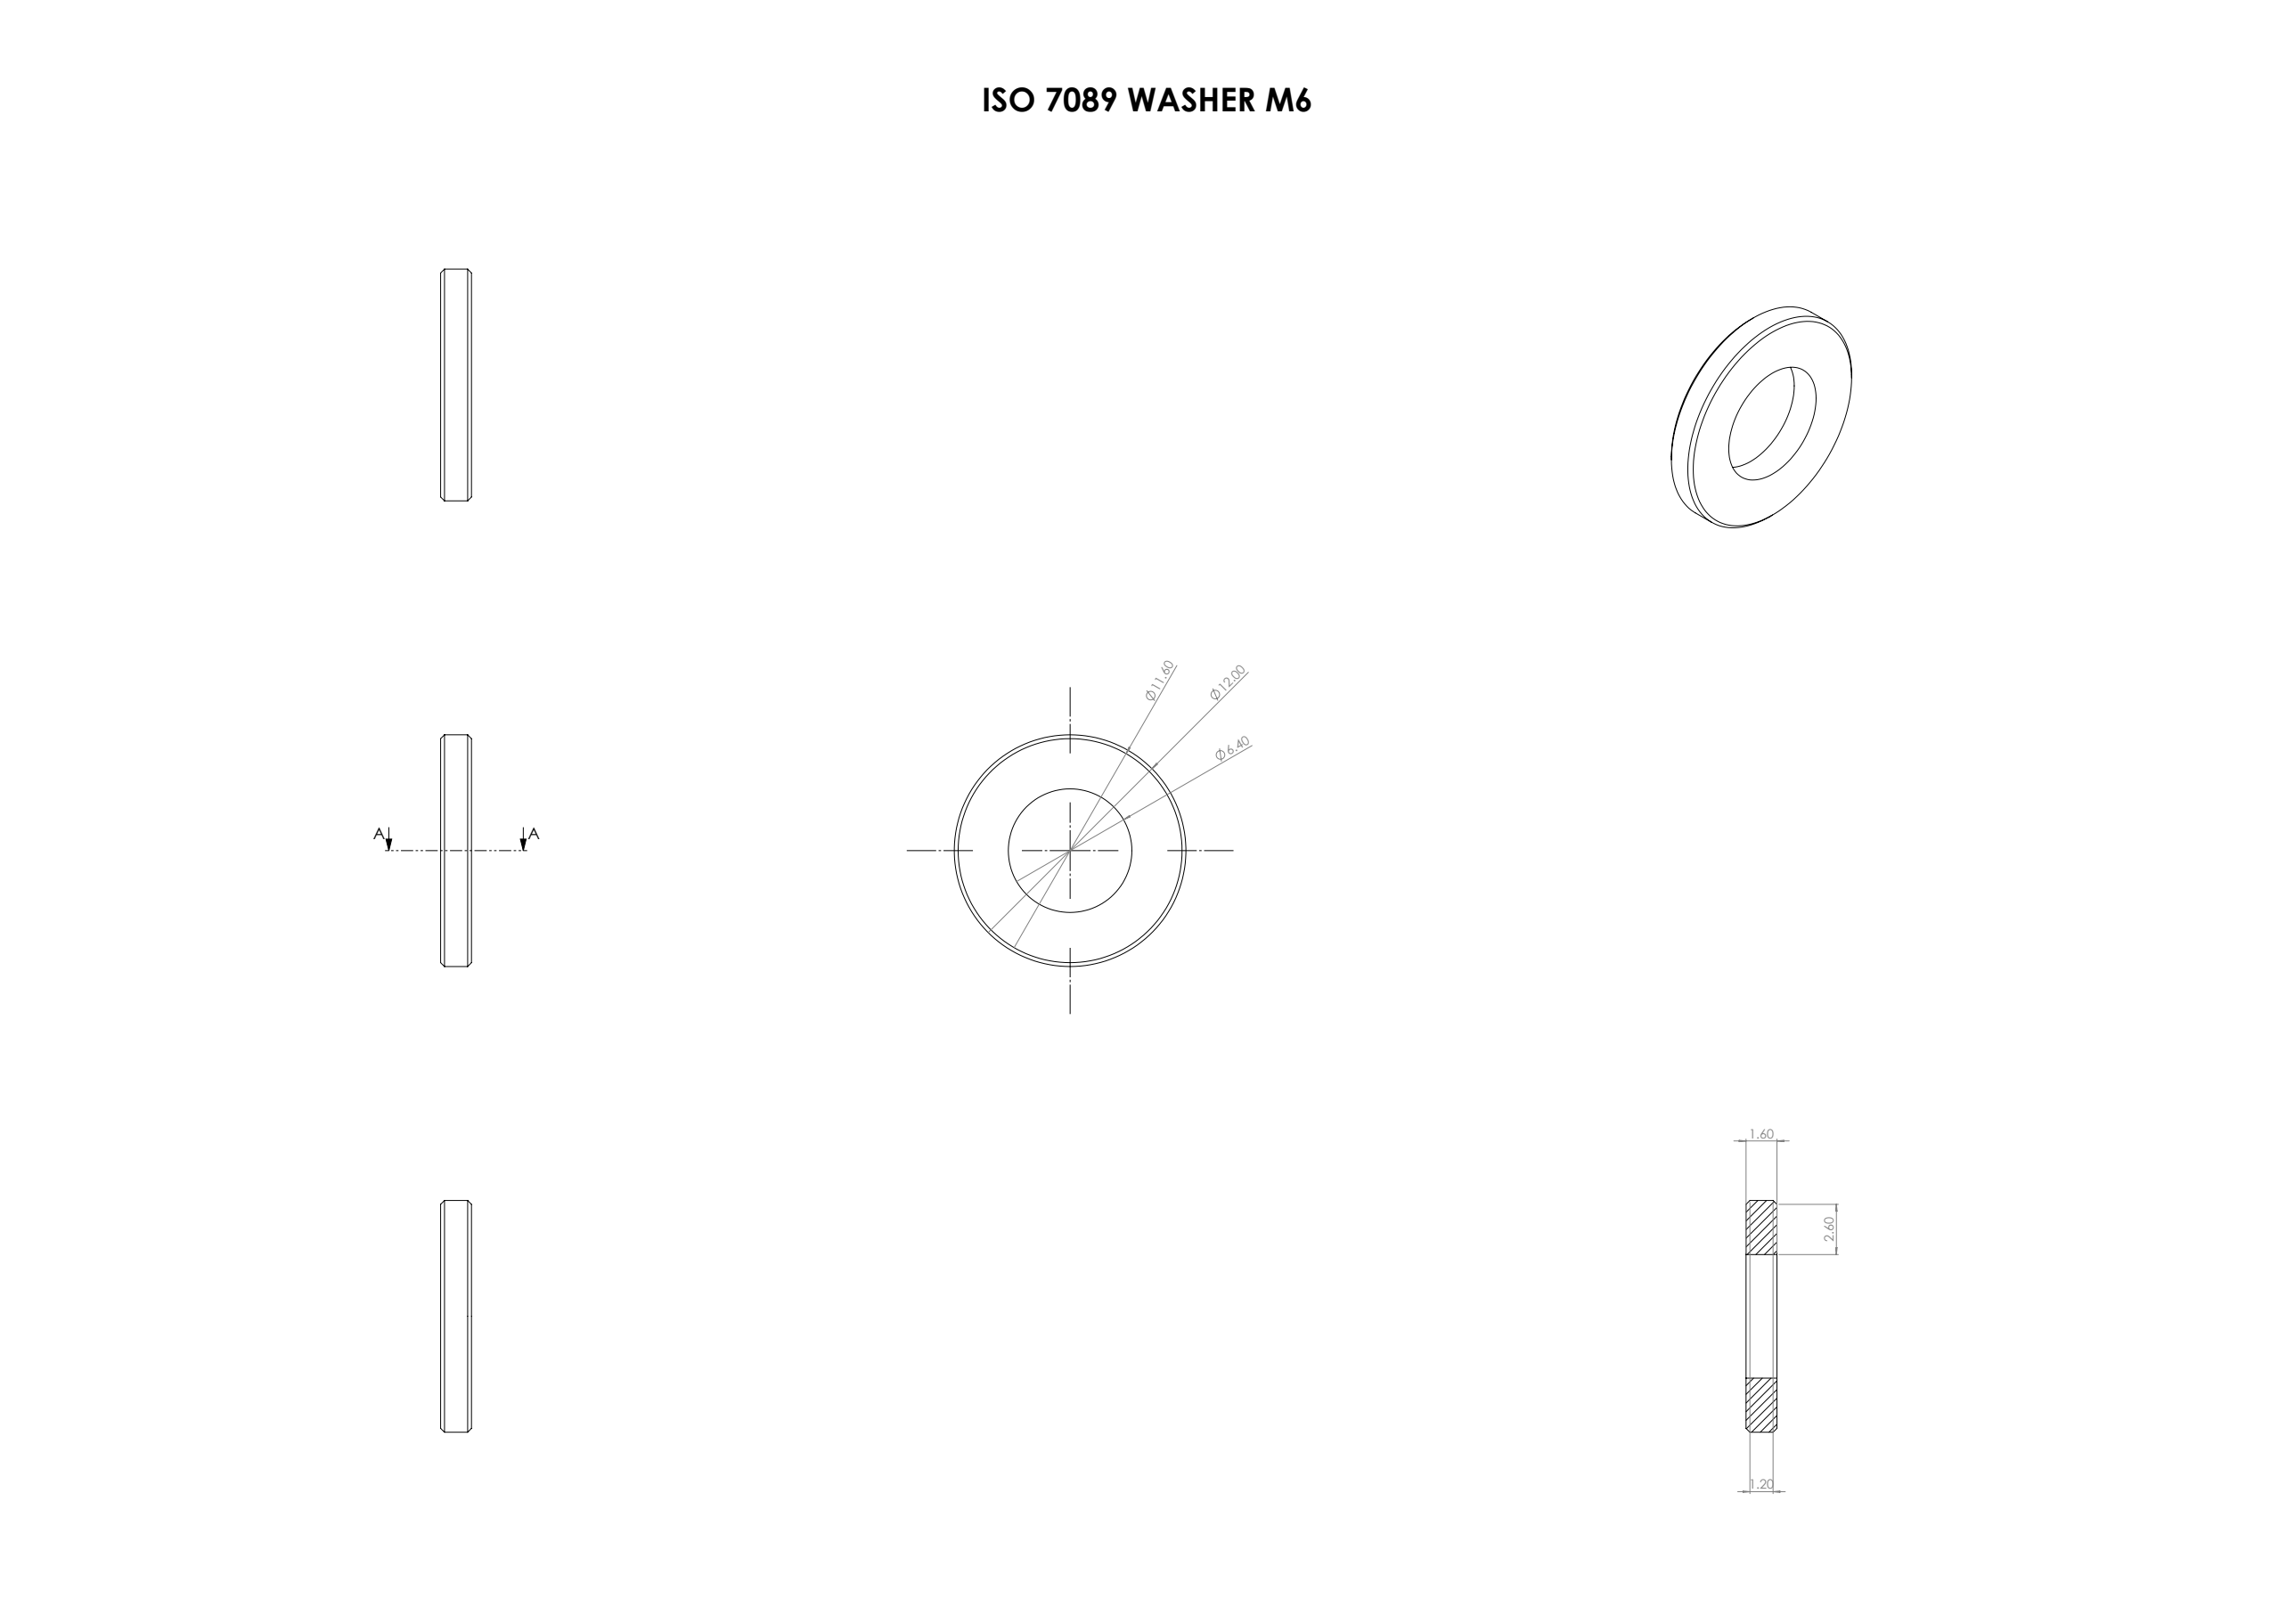
ISO-10303-21;
HEADER;
/* Generated by software containing ST-Developer
 * from STEP Tools, Inc. (www.steptools.com) 
 */

FILE_DESCRIPTION(
/* description */ (''),
/* implementation_level */ '2;1');

FILE_NAME(
/* name */ '07_ISO_7089_Washer_M6.step',
/* time_stamp */ '2026-10-21T02:03:06-07:00',
/* author */ (''),
/* organization */ (''),
/* preprocessor_version */ 'ST-DEVELOPER v20.2',
/* originating_system */ 'Autodesk Translation Framework v15.15.0.0',
/* authorisation */ '');

FILE_SCHEMA (('AUTOMOTIVE_DESIGN { 1 0 10303 214 3 1 1 }'));
ENDSEC;

DATA;
#10=MECHANICAL_DESIGN_GEOMETRIC_PRESENTATION_REPRESENTATION('',(#121),#38528);
#97=SHAPE_REPRESENTATION_RELATIONSHIP('SRR','None',#38582,#109);
#109=ADVANCED_BREP_SHAPE_REPRESENTATION('',(#133),#38522);
#121=STYLED_ITEM('',(#38713),#133);
#133=MANIFOLD_SOLID_BREP('Body1',#17078);
#383=CYLINDRICAL_SURFACE('',#18713,6.);
#384=CYLINDRICAL_SURFACE('',#18717,3.2);
#1034=CONICAL_SURFACE('',#18709,5.9,0.785398163397449);
#1035=CONICAL_SURFACE('',#18721,5.9,0.785398163397449);
#1471=FACE_BOUND('',#4085,.T.);
#1472=FACE_BOUND('',#4088,.T.);
#2177=CIRCLE('',#18710,5.8);
#2178=CIRCLE('',#18711,6.);
#2179=CIRCLE('',#18712,6.);
#2180=CIRCLE('',#18714,6.);
#2181=CIRCLE('',#18716,3.2);
#2182=CIRCLE('',#18718,3.2);
#2183=CIRCLE('',#18720,5.8);
#3060=FACE_OUTER_BOUND('',#4082,.T.);
#3061=FACE_OUTER_BOUND('',#4083,.T.);
#3062=FACE_OUTER_BOUND('',#4084,.T.);
#3063=FACE_OUTER_BOUND('',#4086,.T.);
#3064=FACE_OUTER_BOUND('',#4087,.T.);
#3065=FACE_OUTER_BOUND('',#4089,.T.);
#4082=EDGE_LOOP('',(#14531,#14532,#14533,#14534,#14535));
#4083=EDGE_LOOP('',(#14536,#14537,#14538,#14539,#14540));
#4084=EDGE_LOOP('',(#14541));
#4085=EDGE_LOOP('',(#14542));
#4086=EDGE_LOOP('',(#14543,#14544,#14545,#14546));
#4087=EDGE_LOOP('',(#14547));
#4088=EDGE_LOOP('',(#14548));
#4089=EDGE_LOOP('',(#14549,#14550,#14551,#14552));
#5028=LINE('',#33185,#6003);
#5029=LINE('',#33191,#6004);
#5030=LINE('',#33198,#6005);
#5031=LINE('',#33204,#6006);
#6003=VECTOR('',#22750,5.9);
#6004=VECTOR('',#22757,6.);
#6005=VECTOR('',#22766,3.2);
#6006=VECTOR('',#22775,5.9);
#7528=VERTEX_POINT('',#33182);
#7529=VERTEX_POINT('',#33184);
#7530=VERTEX_POINT('',#33186);
#7531=VERTEX_POINT('',#33190);
#7532=VERTEX_POINT('',#33194);
#7533=VERTEX_POINT('',#33197);
#7534=VERTEX_POINT('',#33201);
#9917=EDGE_CURVE('',#7528,#7528,#2177,.T.);
#9918=EDGE_CURVE('',#7528,#7529,#5028,.T.);
#9919=EDGE_CURVE('',#7529,#7530,#2178,.T.);
#9920=EDGE_CURVE('',#7530,#7529,#2179,.T.);
#9921=EDGE_CURVE('',#7530,#7531,#5029,.T.);
#9922=EDGE_CURVE('',#7531,#7531,#2180,.T.);
#9923=EDGE_CURVE('',#7532,#7532,#2181,.T.);
#9924=EDGE_CURVE('',#7532,#7533,#5030,.T.);
#9925=EDGE_CURVE('',#7533,#7533,#2182,.T.);
#9926=EDGE_CURVE('',#7534,#7534,#2183,.T.);
#9927=EDGE_CURVE('',#7531,#7534,#5031,.T.);
#14531=ORIENTED_EDGE('',*,*,#9917,.T.);
#14532=ORIENTED_EDGE('',*,*,#9918,.T.);
#14533=ORIENTED_EDGE('',*,*,#9919,.T.);
#14534=ORIENTED_EDGE('',*,*,#9920,.T.);
#14535=ORIENTED_EDGE('',*,*,#9918,.F.);
#14536=ORIENTED_EDGE('',*,*,#9919,.F.);
#14537=ORIENTED_EDGE('',*,*,#9920,.F.);
#14538=ORIENTED_EDGE('',*,*,#9921,.T.);
#14539=ORIENTED_EDGE('',*,*,#9922,.T.);
#14540=ORIENTED_EDGE('',*,*,#9921,.F.);
#14541=ORIENTED_EDGE('',*,*,#9917,.F.);
#14542=ORIENTED_EDGE('',*,*,#9923,.F.);
#14543=ORIENTED_EDGE('',*,*,#9923,.T.);
#14544=ORIENTED_EDGE('',*,*,#9924,.T.);
#14545=ORIENTED_EDGE('',*,*,#9925,.F.);
#14546=ORIENTED_EDGE('',*,*,#9924,.F.);
#14547=ORIENTED_EDGE('',*,*,#9926,.F.);
#14548=ORIENTED_EDGE('',*,*,#9925,.T.);
#14549=ORIENTED_EDGE('',*,*,#9922,.F.);
#14550=ORIENTED_EDGE('',*,*,#9927,.T.);
#14551=ORIENTED_EDGE('',*,*,#9926,.T.);
#14552=ORIENTED_EDGE('',*,*,#9927,.F.);
#15960=PLANE('',#18715);
#15961=PLANE('',#18719);
#16869=ADVANCED_FACE('',(#3060),#1034,.T.);
#16870=ADVANCED_FACE('',(#3061),#383,.T.);
#16871=ADVANCED_FACE('',(#3062,#1471),#15960,.T.);
#16872=ADVANCED_FACE('',(#3063),#384,.F.);
#16873=ADVANCED_FACE('',(#3064,#1472),#15961,.T.);
#16874=ADVANCED_FACE('',(#3065),#1035,.T.);
#17078=CLOSED_SHELL('',(#16869,#16870,#16871,#16872,#16873,#16874));
#18708=AXIS2_PLACEMENT_3D('',#33180,#22744,#22745);
#18709=AXIS2_PLACEMENT_3D('',#33181,#22746,#22747);
#18710=AXIS2_PLACEMENT_3D('',#33183,#22748,#22749);
#18711=AXIS2_PLACEMENT_3D('',#33187,#22751,#22752);
#18712=AXIS2_PLACEMENT_3D('',#33188,#22753,#22754);
#18713=AXIS2_PLACEMENT_3D('',#33189,#22755,#22756);
#18714=AXIS2_PLACEMENT_3D('',#33192,#22758,#22759);
#18715=AXIS2_PLACEMENT_3D('',#33193,#22760,#22761);
#18716=AXIS2_PLACEMENT_3D('',#33195,#22762,#22763);
#18717=AXIS2_PLACEMENT_3D('',#33196,#22764,#22765);
#18718=AXIS2_PLACEMENT_3D('',#33199,#22767,#22768);
#18719=AXIS2_PLACEMENT_3D('',#33200,#22769,#22770);
#18720=AXIS2_PLACEMENT_3D('',#33202,#22771,#22772);
#18721=AXIS2_PLACEMENT_3D('',#33203,#22773,#22774);
#22744=DIRECTION('axis',(0.,0.,1.));
#22745=DIRECTION('refdir',(1.,0.,0.));
#22746=DIRECTION('center_axis',(-1.,0.,0.));
#22747=DIRECTION('ref_axis',(0.,-1.,0.));
#22748=DIRECTION('center_axis',(-1.,0.,0.));
#22749=DIRECTION('ref_axis',(0.,-1.,0.));
#22750=DIRECTION('',(-0.707106781186547,0.707106781186548,8.65956056235494E-17));
#22751=DIRECTION('center_axis',(1.,0.,0.));
#22752=DIRECTION('ref_axis',(0.,-1.,0.));
#22753=DIRECTION('center_axis',(1.,0.,0.));
#22754=DIRECTION('ref_axis',(0.,-1.,0.));
#22755=DIRECTION('center_axis',(1.,0.,0.));
#22756=DIRECTION('ref_axis',(0.,1.,0.));
#22757=DIRECTION('',(-1.,0.,0.));
#22758=DIRECTION('center_axis',(1.,0.,0.));
#22759=DIRECTION('ref_axis',(0.,0.,-1.));
#22760=DIRECTION('center_axis',(1.,0.,0.));
#22761=DIRECTION('ref_axis',(0.,0.,-1.));
#22762=DIRECTION('center_axis',(1.,0.,0.));
#22763=DIRECTION('ref_axis',(0.,0.,-1.));
#22764=DIRECTION('center_axis',(1.,0.,0.));
#22765=DIRECTION('ref_axis',(0.,1.,0.));
#22766=DIRECTION('',(-1.,0.,0.));
#22767=DIRECTION('center_axis',(1.,0.,0.));
#22768=DIRECTION('ref_axis',(0.,0.,-1.));
#22769=DIRECTION('center_axis',(-1.,0.,0.));
#22770=DIRECTION('ref_axis',(0.,0.,1.));
#22771=DIRECTION('center_axis',(1.,0.,0.));
#22772=DIRECTION('ref_axis',(0.,0.,-1.));
#22773=DIRECTION('center_axis',(1.,0.,0.));
#22774=DIRECTION('ref_axis',(0.,1.,0.));
#22775=DIRECTION('',(-0.707106781186547,0.707106781186548,8.65956056235494E-17));
#33180=CARTESIAN_POINT('',(0.,0.,0.));
#33181=CARTESIAN_POINT('Origin',(1.5,0.,0.));
#33182=CARTESIAN_POINT('',(1.6,5.8,-7.10295143505465E-16));
#33183=CARTESIAN_POINT('Origin',(1.6,0.,0.));
#33184=CARTESIAN_POINT('',(1.4,6.,7.34788079488412E-16));
#33185=CARTESIAN_POINT('',(1.5,5.9,7.22541611496938E-16));
#33186=CARTESIAN_POINT('',(1.4,-6.,-7.34788079488412E-16));
#33187=CARTESIAN_POINT('Origin',(1.4,0.,0.));
#33188=CARTESIAN_POINT('Origin',(1.4,0.,0.));
#33189=CARTESIAN_POINT('Origin',(0.9,0.,0.));
#33190=CARTESIAN_POINT('',(0.2,-6.,-7.34788079488412E-16));
#33191=CARTESIAN_POINT('',(0.9,-6.,-7.34788079488412E-16));
#33192=CARTESIAN_POINT('Origin',(0.2,0.,0.));
#33193=CARTESIAN_POINT('Origin',(1.6,3.2,0.));
#33194=CARTESIAN_POINT('',(1.6,-3.2,-3.91886975727153E-16));
#33195=CARTESIAN_POINT('Origin',(1.6,0.,0.));
#33196=CARTESIAN_POINT('Origin',(0.8,0.,0.));
#33197=CARTESIAN_POINT('',(0.,-3.2,-3.91886975727153E-16));
#33198=CARTESIAN_POINT('',(0.8,-3.2,-3.91886975727153E-16));
#33199=CARTESIAN_POINT('Origin',(0.,0.,0.));
#33200=CARTESIAN_POINT('Origin',(0.,5.8,0.));
#33201=CARTESIAN_POINT('',(-1.21430643318376E-16,-5.8,-7.10295143505465E-16));
#33202=CARTESIAN_POINT('Origin',(0.,0.,0.));
#33203=CARTESIAN_POINT('Origin',(0.1,0.,0.));
#33204=CARTESIAN_POINT('',(0.1,-5.9,-7.22541611496938E-16));
#38508=UNCERTAINTY_MEASURE_WITH_UNIT(LENGTH_MEASURE(0.01),#38529,
'DISTANCE_ACCURACY_VALUE',
'Maximum model space distance between geometric entities at asserted c
onnectivities');
#38514=UNCERTAINTY_MEASURE_WITH_UNIT(LENGTH_MEASURE(0.01),#38529,
'DISTANCE_ACCURACY_VALUE',
'Maximum model space distance between geometric entities at asserted c
onnectivities');
#38522=(
GEOMETRIC_REPRESENTATION_CONTEXT(3)
GLOBAL_UNCERTAINTY_ASSIGNED_CONTEXT((#38508))
GLOBAL_UNIT_ASSIGNED_CONTEXT((#38529,#38531,#38532))
REPRESENTATION_CONTEXT('','3D')
);
#38528=(
GEOMETRIC_REPRESENTATION_CONTEXT(3)
GLOBAL_UNCERTAINTY_ASSIGNED_CONTEXT((#38514))
GLOBAL_UNIT_ASSIGNED_CONTEXT((#38529,#38531,#38532))
REPRESENTATION_CONTEXT('','3D')
);
#38529=(
LENGTH_UNIT()
NAMED_UNIT(*)
SI_UNIT(.MILLI.,.METRE.)
);
#38531=(
NAMED_UNIT(*)
PLANE_ANGLE_UNIT()
SI_UNIT($,.RADIAN.)
);
#38532=(
NAMED_UNIT(*)
SI_UNIT($,.STERADIAN.)
SOLID_ANGLE_UNIT()
);
#38540=SHAPE_DEFINITION_REPRESENTATION(#38553,#38582);
#38553=PRODUCT_DEFINITION_SHAPE('',$,#38596);
#38582=SHAPE_REPRESENTATION('',(#18708),#38522);
#38588=PRODUCT_DEFINITION_CONTEXT('part definition',#38629,'design');
#38596=PRODUCT_DEFINITION('2026-10-20-13-39-09-288',
'07_ISO_7089_Washer_M6',#38609,#38588);
#38609=PRODUCT_DEFINITION_FORMATION('',$,#38638);
#38629=APPLICATION_CONTEXT(
'Core Data for Automotive Mechanical Design Process');
#38630=PRODUCT_CONTEXT('part definition',#38629,'mechanical');
#38638=PRODUCT('2026-10-20-13-39-09-288','07_ISO_7089_Washer_M6',$,(#38630));
#38707=COLOUR_RGB('Black',0.12,0.14,0.17);
#38708=FILL_AREA_STYLE_COLOUR('',#38707);
#38709=FILL_AREA_STYLE('',(#38708));
#38710=SURFACE_STYLE_FILL_AREA(#38709);
#38711=SURFACE_SIDE_STYLE('',(#38710));
#38712=SURFACE_STYLE_USAGE(.BOTH.,#38711);
#38713=PRESENTATION_STYLE_ASSIGNMENT((#38712));
ENDSEC;
END-ISO-10303-21;
